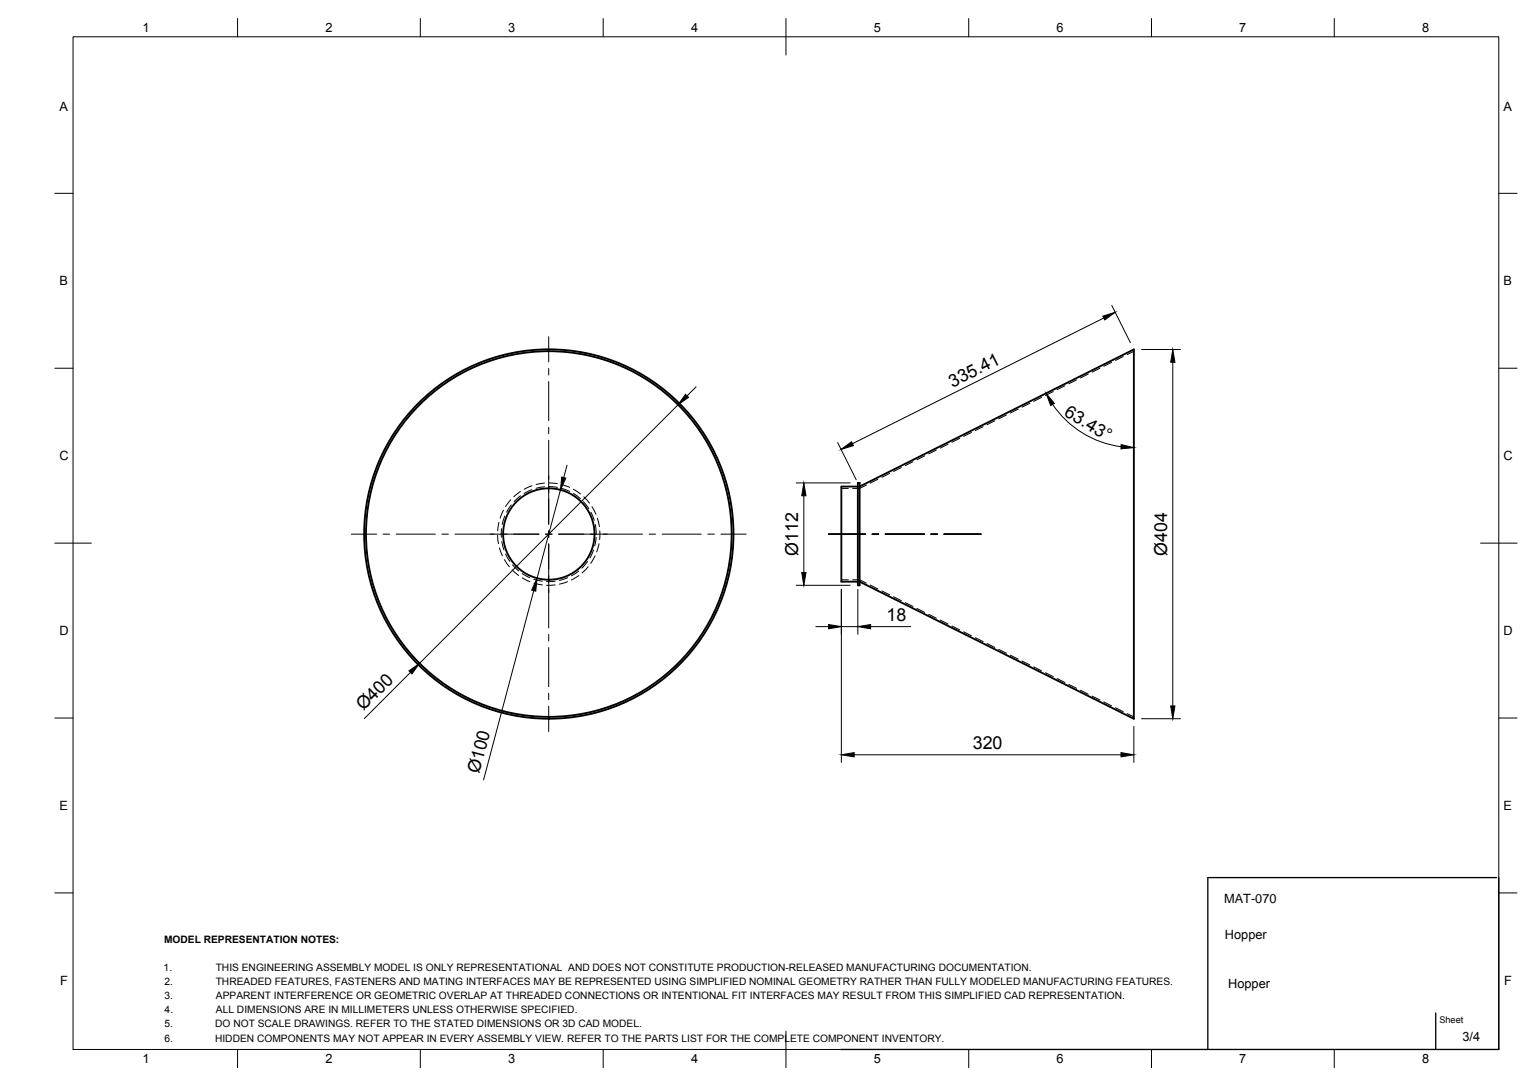
ISO-10303-21;
HEADER;
/* Generated by software containing ST-Developer
 * from STEP Tools, Inc. (www.steptools.com) 
 */

FILE_DESCRIPTION(
/* description */ (''),
/* implementation_level */ '2;1');

FILE_NAME(
/* name */ 'Hopper.step',
/* time_stamp */ '2026-10-24T12:18:10-07:00',
/* author */ (''),
/* organization */ (''),
/* preprocessor_version */ 'ST-DEVELOPER v20.2',
/* originating_system */ 'Autodesk Translation Framework v15.15.0.0',
/* authorisation */ '');

FILE_SCHEMA (('AUTOMOTIVE_DESIGN { 1 0 10303 214 3 1 1 }'));
ENDSEC;

DATA;
#10=MECHANICAL_DESIGN_GEOMETRIC_PRESENTATION_REPRESENTATION('',(#38),#2858);
#34=SHAPE_REPRESENTATION_RELATIONSHIP('SRR','None',#2872,#36);
#36=ADVANCED_BREP_SHAPE_REPRESENTATION('',(#40),#2856);
#38=STYLED_ITEM('',(#2890),#40);
#40=MANIFOLD_SOLID_BREP('Hopper',#389);
#42=CYLINDRICAL_SURFACE('',#423,50.);
#43=CYLINDRICAL_SURFACE('',#425,52.);
#44=CYLINDRICAL_SURFACE('',#429,56.);
#49=LINE('',#569,#72);
#50=LINE('',#574,#73);
#51=LINE('',#578,#74);
#52=LINE('',#583,#75);
#53=LINE('',#590,#76);
#72=VECTOR('',#467,52.);
#73=VECTOR('',#474,200.);
#74=VECTOR('',#479,50.);
#75=VECTOR('',#484,52.);
#76=VECTOR('',#493,56.);
#95=CONICAL_SURFACE('',#419,52.,0.463647609000806);
#96=CONICAL_SURFACE('',#421,200.,0.463647609000806);
#97=FACE_BOUND('',#127,.T.);
#98=FACE_BOUND('',#133,.T.);
#99=FACE_BOUND('',#136,.T.);
#100=FACE_BOUND('',#138,.T.);
#102=FACE_OUTER_BOUND('',#126,.T.);
#103=FACE_OUTER_BOUND('',#128,.T.);
#104=FACE_OUTER_BOUND('',#129,.T.);
#105=FACE_OUTER_BOUND('',#130,.T.);
#106=FACE_OUTER_BOUND('',#131,.T.);
#107=FACE_OUTER_BOUND('',#132,.T.);
#108=FACE_OUTER_BOUND('',#134,.T.);
#109=FACE_OUTER_BOUND('',#135,.T.);
#110=FACE_OUTER_BOUND('',#137,.T.);
#126=EDGE_LOOP('',(#253));
#127=EDGE_LOOP('',(#254));
#128=EDGE_LOOP('',(#255,#256,#257,#258));
#129=EDGE_LOOP('',(#259,#260,#261,#262));
#130=EDGE_LOOP('',(#263,#264,#265,#266));
#131=EDGE_LOOP('',(#267,#268,#269,#270));
#132=EDGE_LOOP('',(#271));
#133=EDGE_LOOP('',(#272));
#134=EDGE_LOOP('',(#273,#274,#275,#276));
#135=EDGE_LOOP('',(#277));
#136=EDGE_LOOP('',(#278));
#137=EDGE_LOOP('',(#279));
#138=EDGE_LOOP('',(#280));
#155=CIRCLE('',#417,202.);
#156=CIRCLE('',#418,200.);
#157=CIRCLE('',#420,52.);
#158=CIRCLE('',#422,50.);
#159=CIRCLE('',#424,50.);
#160=CIRCLE('',#426,52.);
#161=CIRCLE('',#427,52.);
#162=CIRCLE('',#430,56.);
#163=CIRCLE('',#431,56.);
#170=VERTEX_POINT('',#563);
#171=VERTEX_POINT('',#565);
#172=VERTEX_POINT('',#568);
#173=VERTEX_POINT('',#572);
#174=VERTEX_POINT('',#576);
#175=VERTEX_POINT('',#580);
#176=VERTEX_POINT('',#582);
#177=VERTEX_POINT('',#587);
#178=VERTEX_POINT('',#589);
#203=EDGE_CURVE('',#170,#170,#155,.T.);
#204=EDGE_CURVE('',#171,#171,#156,.T.);
#205=EDGE_CURVE('',#170,#172,#49,.T.);
#206=EDGE_CURVE('',#172,#172,#157,.T.);
#207=EDGE_CURVE('',#173,#173,#158,.T.);
#208=EDGE_CURVE('',#173,#171,#50,.T.);
#209=EDGE_CURVE('',#174,#174,#159,.F.);
#210=EDGE_CURVE('',#174,#173,#51,.T.);
#211=EDGE_CURVE('',#175,#175,#160,.T.);
#212=EDGE_CURVE('',#175,#176,#52,.T.);
#213=EDGE_CURVE('',#176,#176,#161,.T.);
#214=EDGE_CURVE('',#177,#177,#162,.T.);
#215=EDGE_CURVE('',#177,#178,#53,.T.);
#216=EDGE_CURVE('',#178,#178,#163,.T.);
#253=ORIENTED_EDGE('',*,*,#203,.T.);
#254=ORIENTED_EDGE('',*,*,#204,.F.);
#255=ORIENTED_EDGE('',*,*,#203,.F.);
#256=ORIENTED_EDGE('',*,*,#205,.T.);
#257=ORIENTED_EDGE('',*,*,#206,.F.);
#258=ORIENTED_EDGE('',*,*,#205,.F.);
#259=ORIENTED_EDGE('',*,*,#207,.F.);
#260=ORIENTED_EDGE('',*,*,#208,.T.);
#261=ORIENTED_EDGE('',*,*,#204,.T.);
#262=ORIENTED_EDGE('',*,*,#208,.F.);
#263=ORIENTED_EDGE('',*,*,#209,.F.);
#264=ORIENTED_EDGE('',*,*,#210,.T.);
#265=ORIENTED_EDGE('',*,*,#207,.T.);
#266=ORIENTED_EDGE('',*,*,#210,.F.);
#267=ORIENTED_EDGE('',*,*,#211,.T.);
#268=ORIENTED_EDGE('',*,*,#212,.T.);
#269=ORIENTED_EDGE('',*,*,#213,.F.);
#270=ORIENTED_EDGE('',*,*,#212,.F.);
#271=ORIENTED_EDGE('',*,*,#213,.T.);
#272=ORIENTED_EDGE('',*,*,#209,.T.);
#273=ORIENTED_EDGE('',*,*,#214,.T.);
#274=ORIENTED_EDGE('',*,*,#215,.T.);
#275=ORIENTED_EDGE('',*,*,#216,.F.);
#276=ORIENTED_EDGE('',*,*,#215,.F.);
#277=ORIENTED_EDGE('',*,*,#216,.T.);
#278=ORIENTED_EDGE('',*,*,#211,.F.);
#279=ORIENTED_EDGE('',*,*,#214,.F.);
#280=ORIENTED_EDGE('',*,*,#206,.T.);
#353=PLANE('',#416);
#354=PLANE('',#428);
#355=PLANE('',#432);
#356=PLANE('',#433);
#365=ADVANCED_FACE('',(#102,#97),#353,.F.);
#366=ADVANCED_FACE('',(#103),#95,.T.);
#367=ADVANCED_FACE('',(#104),#96,.F.);
#368=ADVANCED_FACE('',(#105),#42,.F.);
#369=ADVANCED_FACE('',(#106),#43,.T.);
#370=ADVANCED_FACE('',(#107,#98),#354,.T.);
#371=ADVANCED_FACE('',(#108),#44,.T.);
#372=ADVANCED_FACE('',(#109,#99),#355,.T.);
#373=ADVANCED_FACE('',(#110,#100),#356,.F.);
#389=CLOSED_SHELL('',(#365,#366,#367,#368,#369,#370,#371,#372,#373));
#415=AXIS2_PLACEMENT_3D('',#561,#457,#458);
#416=AXIS2_PLACEMENT_3D('',#562,#459,#460);
#417=AXIS2_PLACEMENT_3D('',#564,#461,#462);
#418=AXIS2_PLACEMENT_3D('',#566,#463,#464);
#419=AXIS2_PLACEMENT_3D('',#567,#465,#466);
#420=AXIS2_PLACEMENT_3D('',#570,#468,#469);
#421=AXIS2_PLACEMENT_3D('',#571,#470,#471);
#422=AXIS2_PLACEMENT_3D('',#573,#472,#473);
#423=AXIS2_PLACEMENT_3D('',#575,#475,#476);
#424=AXIS2_PLACEMENT_3D('',#577,#477,#478);
#425=AXIS2_PLACEMENT_3D('',#579,#480,#481);
#426=AXIS2_PLACEMENT_3D('',#581,#482,#483);
#427=AXIS2_PLACEMENT_3D('',#584,#485,#486);
#428=AXIS2_PLACEMENT_3D('',#585,#487,#488);
#429=AXIS2_PLACEMENT_3D('',#586,#489,#490);
#430=AXIS2_PLACEMENT_3D('',#588,#491,#492);
#431=AXIS2_PLACEMENT_3D('',#591,#494,#495);
#432=AXIS2_PLACEMENT_3D('',#592,#496,#497);
#433=AXIS2_PLACEMENT_3D('',#593,#498,#499);
#457=DIRECTION('axis',(0.,0.,1.));
#458=DIRECTION('refdir',(1.,0.,0.));
#459=DIRECTION('center_axis',(0.,-1.,0.));
#460=DIRECTION('ref_axis',(0.,0.,-1.));
#461=DIRECTION('center_axis',(0.,1.,0.));
#462=DIRECTION('ref_axis',(0.,0.,1.));
#463=DIRECTION('center_axis',(0.,1.,0.));
#464=DIRECTION('ref_axis',(0.,0.,1.));
#465=DIRECTION('center_axis',(0.,1.,0.));
#466=DIRECTION('ref_axis',(0.,0.,1.));
#467=DIRECTION('',(5.47678698264202E-17,-0.894427190999916,0.447213595499958));
#468=DIRECTION('center_axis',(0.,-1.,0.));
#469=DIRECTION('ref_axis',(0.,0.,-1.));
#470=DIRECTION('center_axis',(0.,1.,0.));
#471=DIRECTION('ref_axis',(0.,0.,1.));
#472=DIRECTION('center_axis',(0.,1.,0.));
#473=DIRECTION('ref_axis',(0.,0.,1.));
#474=DIRECTION('',(-5.47678698264202E-17,0.894427190999916,-0.447213595499958));
#475=DIRECTION('center_axis',(0.,1.,0.));
#476=DIRECTION('ref_axis',(0.,0.,1.));
#477=DIRECTION('center_axis',(0.,-1.,0.));
#478=DIRECTION('ref_axis',(0.,0.,-1.));
#479=DIRECTION('',(0.,1.,0.));
#480=DIRECTION('center_axis',(0.,1.,0.));
#481=DIRECTION('ref_axis',(0.,0.,1.));
#482=DIRECTION('center_axis',(0.,-1.,0.));
#483=DIRECTION('ref_axis',(0.,0.,-1.));
#484=DIRECTION('',(0.,-1.,0.));
#485=DIRECTION('center_axis',(0.,-1.,0.));
#486=DIRECTION('ref_axis',(0.,0.,-1.));
#487=DIRECTION('center_axis',(0.,-1.,0.));
#488=DIRECTION('ref_axis',(0.,0.,-1.));
#489=DIRECTION('center_axis',(0.,1.,0.));
#490=DIRECTION('ref_axis',(0.,0.,1.));
#491=DIRECTION('center_axis',(0.,-1.,0.));
#492=DIRECTION('ref_axis',(0.,0.,-1.));
#493=DIRECTION('',(0.,-1.,0.));
#494=DIRECTION('center_axis',(0.,-1.,0.));
#495=DIRECTION('ref_axis',(0.,0.,-1.));
#496=DIRECTION('center_axis',(0.,-1.,0.));
#497=DIRECTION('ref_axis',(0.,0.,-1.));
#498=DIRECTION('center_axis',(0.,-1.,0.));
#499=DIRECTION('ref_axis',(0.,0.,-1.));
#561=CARTESIAN_POINT('',(0.,0.,0.));
#562=CARTESIAN_POINT('Origin',(200.,150.,0.));
#563=CARTESIAN_POINT('',(-2.47378653427765E-14,150.,-202.));
#564=CARTESIAN_POINT('Origin',(0.,150.,0.));
#565=CARTESIAN_POINT('',(-2.44929359829471E-14,150.,-200.));
#566=CARTESIAN_POINT('Origin',(0.,150.,0.));
#567=CARTESIAN_POINT('Origin',(0.,-150.,0.));
#568=CARTESIAN_POINT('',(0.,-150.,-52.));
#569=CARTESIAN_POINT('',(-6.36816335556624E-15,-150.,-52.));
#570=CARTESIAN_POINT('Origin',(0.,-150.,0.));
#571=CARTESIAN_POINT('Origin',(0.,150.,0.));
#572=CARTESIAN_POINT('',(-6.12323399573677E-15,-150.,-50.0000000000001));
#573=CARTESIAN_POINT('Origin',(0.,-150.,0.));
#574=CARTESIAN_POINT('',(-2.44929359829471E-14,150.,-200.));
#575=CARTESIAN_POINT('Origin',(0.,-170.,0.));
#576=CARTESIAN_POINT('',(0.,-170.,-50.));
#577=CARTESIAN_POINT('Origin',(0.,-170.,0.));
#578=CARTESIAN_POINT('',(-6.12323399573677E-15,-170.,-50.));
#579=CARTESIAN_POINT('Origin',(0.,-170.,0.));
#580=CARTESIAN_POINT('',(0.,-152.,-52.));
#581=CARTESIAN_POINT('Origin',(0.,-152.,0.));
#582=CARTESIAN_POINT('',(0.,-170.,-52.));
#583=CARTESIAN_POINT('',(-6.36816335556624E-15,-170.,-52.));
#584=CARTESIAN_POINT('Origin',(0.,-170.,0.));
#585=CARTESIAN_POINT('Origin',(0.,-170.,0.));
#586=CARTESIAN_POINT('Origin',(0.,-152.,0.));
#587=CARTESIAN_POINT('',(0.,-150.,-56.));
#588=CARTESIAN_POINT('Origin',(0.,-150.,0.));
#589=CARTESIAN_POINT('',(0.,-152.,-56.));
#590=CARTESIAN_POINT('',(-6.85802207522518E-15,-152.,-56.));
#591=CARTESIAN_POINT('Origin',(0.,-152.,0.));
#592=CARTESIAN_POINT('Origin',(0.,-152.,0.));
#593=CARTESIAN_POINT('Origin',(0.,-150.,0.));
#2852=UNCERTAINTY_MEASURE_WITH_UNIT(LENGTH_MEASURE(0.01),#2859,
'DISTANCE_ACCURACY_VALUE',
'Maximum model space distance between geometric entities at asserted c
onnectivities');
#2854=UNCERTAINTY_MEASURE_WITH_UNIT(LENGTH_MEASURE(0.01),#2859,
'DISTANCE_ACCURACY_VALUE',
'Maximum model space distance between geometric entities at asserted c
onnectivities');
#2856=(
GEOMETRIC_REPRESENTATION_CONTEXT(3)
GLOBAL_UNCERTAINTY_ASSIGNED_CONTEXT((#2852))
GLOBAL_UNIT_ASSIGNED_CONTEXT((#2859,#2861,#2862))
REPRESENTATION_CONTEXT('','3D')
);
#2858=(
GEOMETRIC_REPRESENTATION_CONTEXT(3)
GLOBAL_UNCERTAINTY_ASSIGNED_CONTEXT((#2854))
GLOBAL_UNIT_ASSIGNED_CONTEXT((#2859,#2861,#2862))
REPRESENTATION_CONTEXT('','3D')
);
#2859=(
LENGTH_UNIT()
NAMED_UNIT(*)
SI_UNIT(.MILLI.,.METRE.)
);
#2861=(
NAMED_UNIT(*)
PLANE_ANGLE_UNIT()
SI_UNIT($,.RADIAN.)
);
#2862=(
NAMED_UNIT(*)
SI_UNIT($,.STERADIAN.)
SOLID_ANGLE_UNIT()
);
#2864=SHAPE_DEFINITION_REPRESENTATION(#2867,#2872);
#2867=PRODUCT_DEFINITION_SHAPE('',$,#2876);
#2872=SHAPE_REPRESENTATION('',(#415),#2856);
#2874=PRODUCT_DEFINITION_CONTEXT('part definition',#2885,'design');
#2876=PRODUCT_DEFINITION('Hopper','Hopper',#2879,#2874);
#2879=PRODUCT_DEFINITION_FORMATION('',$,#2888);
#2885=APPLICATION_CONTEXT(
'Core Data for Automotive Mechanical Design Process');
#2886=PRODUCT_CONTEXT('part definition',#2885,'mechanical');
#2888=PRODUCT('Hopper','Hopper',$,(#2886));
#2890=PRESENTATION_STYLE_ASSIGNMENT((#2891));
#2891=SURFACE_STYLE_USAGE(.BOTH.,#2892);
#2892=SURFACE_SIDE_STYLE('',(#2893));
#2893=SURFACE_STYLE_FILL_AREA(#2894);
#2894=FILL_AREA_STYLE('Steel - Satin',(#2895));
#2895=FILL_AREA_STYLE_COLOUR('Steel - Satin',#2896);
#2896=COLOUR_RGB('Steel - Satin',0.627450980392157,0.627450980392157,0.627450980392157);
ENDSEC;
END-ISO-10303-21;
